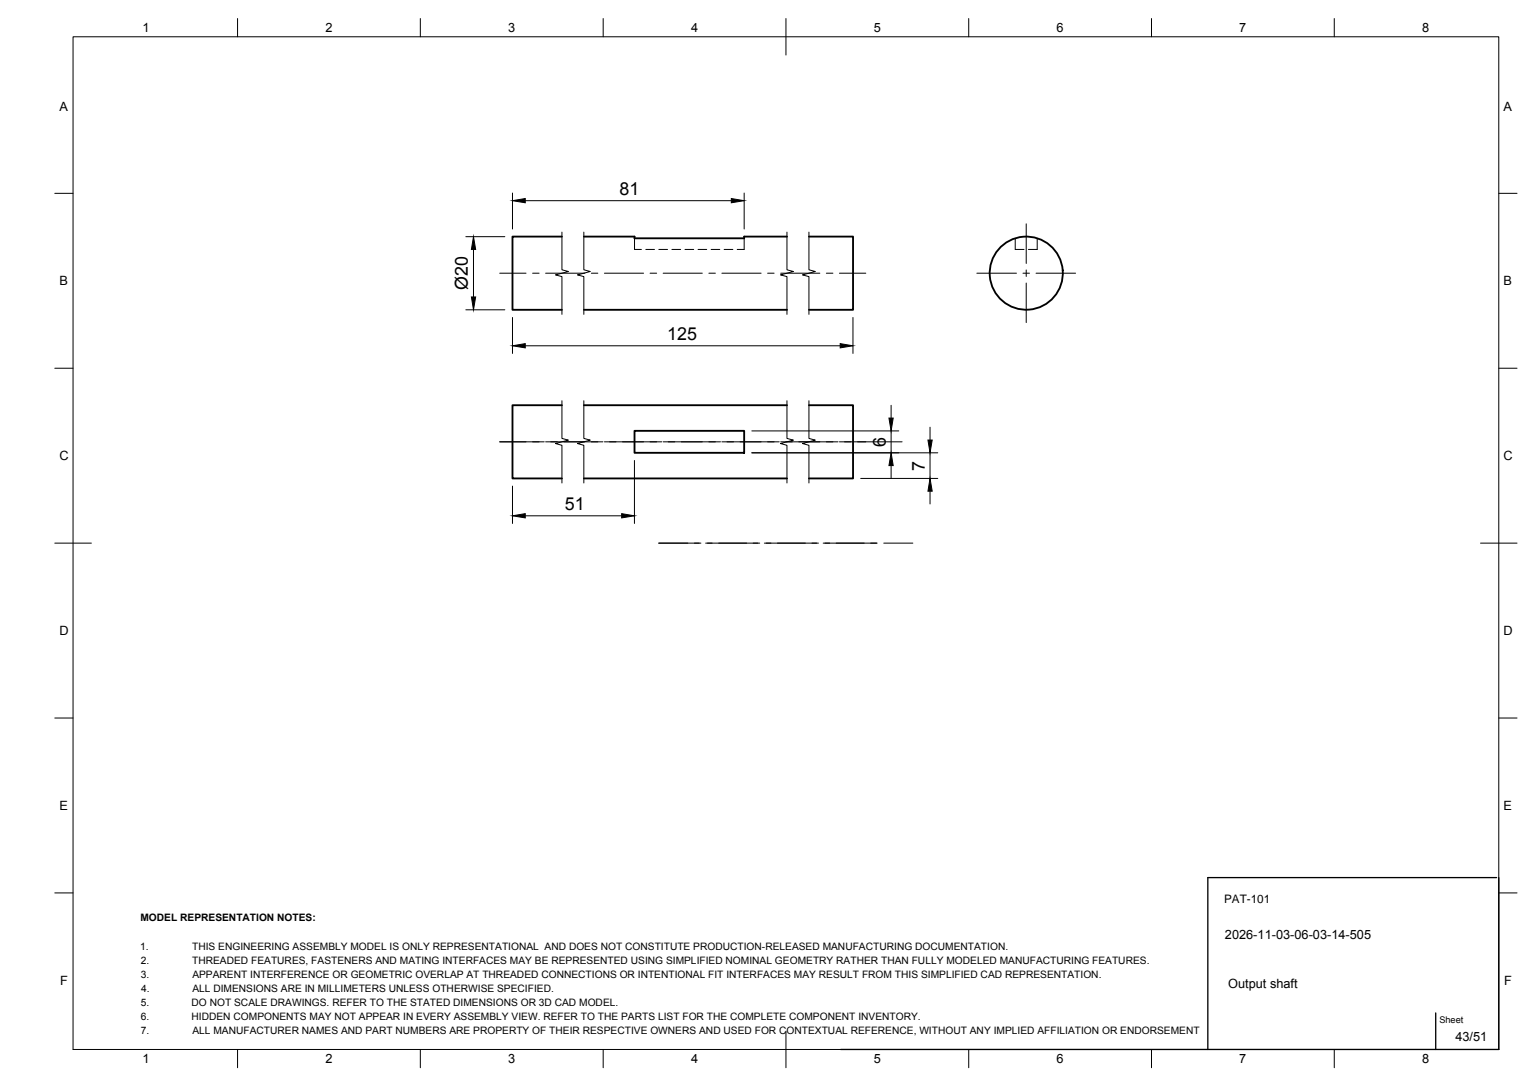
ISO-10303-21;
HEADER;
/* Generated by software containing ST-Developer
 * from STEP Tools, Inc. (www.steptools.com) 
 */

FILE_DESCRIPTION(
/* description */ ('Spur gear reduction stage 2-1 on bearing plates'),
/* implementation_level */ '2;1');

FILE_NAME(
/* name */ 'Output shaft.step',
/* time_stamp */ '2026-10-28T03:22:07-07:00',
/* author */ (''),
/* organization */ (''),
/* preprocessor_version */ 'ST-DEVELOPER v20.2',
/* originating_system */ 'Autodesk Translation Framework v15.17.0.0',
/* authorisation */ '');

FILE_SCHEMA (('AUTOMOTIVE_DESIGN { 1 0 10303 214 3 1 1 }'));
ENDSEC;

DATA;
#10=MECHANICAL_DESIGN_GEOMETRIC_PRESENTATION_REPRESENTATION('',(#995),#53909);
#894=SHAPE_REPRESENTATION_RELATIONSHIP('SRR','None',#54125,#937);
#937=ADVANCED_BREP_SHAPE_REPRESENTATION('',(#1050),#53899);
#995=STYLED_ITEM('',(#54397),#1050);
#1050=MANIFOLD_SOLID_BREP('Body1',#11322);
#1217=FACE_BOUND('',#2734,.T.);
#1415=PLANE('',#12678);
#1416=PLANE('',#12679);
#1417=PLANE('',#12681);
#1418=PLANE('',#12682);
#1419=PLANE('',#12683);
#1420=PLANE('',#12688);
#1421=PLANE('',#12689);
#1923=FACE_OUTER_BOUND('',#2728,.T.);
#1924=FACE_OUTER_BOUND('',#2729,.T.);
#1925=FACE_OUTER_BOUND('',#2730,.T.);
#1926=FACE_OUTER_BOUND('',#2731,.T.);
#1927=FACE_OUTER_BOUND('',#2732,.T.);
#1928=FACE_OUTER_BOUND('',#2733,.T.);
#1929=FACE_OUTER_BOUND('',#2735,.T.);
#1930=FACE_OUTER_BOUND('',#2736,.T.);
#2728=EDGE_LOOP('',(#9190,#9191,#9192,#9193));
#2729=EDGE_LOOP('',(#9194,#9195,#9196,#9197));
#2730=EDGE_LOOP('',(#9198,#9199,#9200,#9201));
#2731=EDGE_LOOP('',(#9202,#9203,#9204,#9205));
#2732=EDGE_LOOP('',(#9206,#9207,#9208,#9209));
#2733=EDGE_LOOP('',(#9210,#9211,#9212,#9213));
#2734=EDGE_LOOP('',(#9214,#9215,#9216,#9217));
#2735=EDGE_LOOP('',(#9218));
#2736=EDGE_LOOP('',(#9219));
#3373=LINE('',#29846,#4014);
#3374=LINE('',#29848,#4015);
#3375=LINE('',#29850,#4016);
#3376=LINE('',#29851,#4017);
#3377=LINE('',#29856,#4018);
#3378=LINE('',#29857,#4019);
#3379=LINE('',#29860,#4020);
#3380=LINE('',#29862,#4021);
#3381=LINE('',#29863,#4022);
#3382=LINE('',#29865,#4023);
#3383=LINE('',#29872,#4024);
#4014=VECTOR('',#15124,1.);
#4015=VECTOR('',#15125,1.);
#4016=VECTOR('',#15126,1.);
#4017=VECTOR('',#15127,1.);
#4018=VECTOR('',#15132,1.);
#4019=VECTOR('',#15133,1.);
#4020=VECTOR('',#15136,1.);
#4021=VECTOR('',#15137,1.);
#4022=VECTOR('',#15138,1.);
#4023=VECTOR('',#15141,1.);
#4024=VECTOR('',#15150,1.);
#4662=CIRCLE('',#12680,1.);
#4663=CIRCLE('',#12684,1.);
#4664=CIRCLE('',#12686,1.);
#4665=CIRCLE('',#12687,1.);
#5408=VERTEX_POINT('',#29844);
#5409=VERTEX_POINT('',#29845);
#5410=VERTEX_POINT('',#29847);
#5411=VERTEX_POINT('',#29849);
#5412=VERTEX_POINT('',#29853);
#5413=VERTEX_POINT('',#29855);
#5414=VERTEX_POINT('',#29859);
#5415=VERTEX_POINT('',#29861);
#5416=VERTEX_POINT('',#29869);
#5417=VERTEX_POINT('',#29871);
#6737=EDGE_CURVE('',#5408,#5409,#3373,.T.);
#6738=EDGE_CURVE('',#5408,#5410,#3374,.T.);
#6739=EDGE_CURVE('',#5411,#5410,#3375,.T.);
#6740=EDGE_CURVE('',#5411,#5409,#3376,.T.);
#6741=EDGE_CURVE('',#5409,#5412,#4662,.T.);
#6742=EDGE_CURVE('',#5413,#5411,#3377,.T.);
#6743=EDGE_CURVE('',#5412,#5413,#3378,.T.);
#6744=EDGE_CURVE('',#5412,#5414,#3379,.T.);
#6745=EDGE_CURVE('',#5413,#5415,#3380,.T.);
#6746=EDGE_CURVE('',#5415,#5414,#3381,.T.);
#6747=EDGE_CURVE('',#5410,#5415,#3382,.T.);
#6748=EDGE_CURVE('',#5414,#5408,#4663,.T.);
#6749=EDGE_CURVE('',#5416,#5416,#4664,.T.);
#6750=EDGE_CURVE('',#5416,#5417,#3383,.T.);
#6751=EDGE_CURVE('',#5417,#5417,#4665,.T.);
#9190=ORIENTED_EDGE('',*,*,#6737,.F.);
#9191=ORIENTED_EDGE('',*,*,#6738,.T.);
#9192=ORIENTED_EDGE('',*,*,#6739,.F.);
#9193=ORIENTED_EDGE('',*,*,#6740,.T.);
#9194=ORIENTED_EDGE('',*,*,#6741,.F.);
#9195=ORIENTED_EDGE('',*,*,#6740,.F.);
#9196=ORIENTED_EDGE('',*,*,#6742,.F.);
#9197=ORIENTED_EDGE('',*,*,#6743,.F.);
#9198=ORIENTED_EDGE('',*,*,#6744,.F.);
#9199=ORIENTED_EDGE('',*,*,#6743,.T.);
#9200=ORIENTED_EDGE('',*,*,#6745,.T.);
#9201=ORIENTED_EDGE('',*,*,#6746,.T.);
#9202=ORIENTED_EDGE('',*,*,#6742,.T.);
#9203=ORIENTED_EDGE('',*,*,#6739,.T.);
#9204=ORIENTED_EDGE('',*,*,#6747,.T.);
#9205=ORIENTED_EDGE('',*,*,#6745,.F.);
#9206=ORIENTED_EDGE('',*,*,#6748,.F.);
#9207=ORIENTED_EDGE('',*,*,#6746,.F.);
#9208=ORIENTED_EDGE('',*,*,#6747,.F.);
#9209=ORIENTED_EDGE('',*,*,#6738,.F.);
#9210=ORIENTED_EDGE('',*,*,#6749,.F.);
#9211=ORIENTED_EDGE('',*,*,#6750,.T.);
#9212=ORIENTED_EDGE('',*,*,#6751,.T.);
#9213=ORIENTED_EDGE('',*,*,#6750,.F.);
#9214=ORIENTED_EDGE('',*,*,#6744,.T.);
#9215=ORIENTED_EDGE('',*,*,#6748,.T.);
#9216=ORIENTED_EDGE('',*,*,#6737,.T.);
#9217=ORIENTED_EDGE('',*,*,#6741,.T.);
#9218=ORIENTED_EDGE('',*,*,#6749,.T.);
#9219=ORIENTED_EDGE('',*,*,#6751,.F.);
#10565=CYLINDRICAL_SURFACE('',#12685,1.);
#11043=ADVANCED_FACE('',(#1923),#1415,.F.);
#11044=ADVANCED_FACE('',(#1924),#1416,.T.);
#11045=ADVANCED_FACE('',(#1925),#1417,.F.);
#11046=ADVANCED_FACE('',(#1926),#1418,.F.);
#11047=ADVANCED_FACE('',(#1927),#1419,.F.);
#11048=ADVANCED_FACE('',(#1928,#1217),#10565,.T.);
#11049=ADVANCED_FACE('',(#1929),#1420,.T.);
#11050=ADVANCED_FACE('',(#1930),#1421,.F.);
#11322=CLOSED_SHELL('',(#11043,#11044,#11045,#11046,#11047,#11048,#11049,
#11050));
#12677=AXIS2_PLACEMENT_3D('',#29842,#15120,#15121);
#12678=AXIS2_PLACEMENT_3D('',#29843,#15122,#15123);
#12679=AXIS2_PLACEMENT_3D('',#29852,#15128,#15129);
#12680=AXIS2_PLACEMENT_3D('',#29854,#15130,#15131);
#12681=AXIS2_PLACEMENT_3D('',#29858,#15134,#15135);
#12682=AXIS2_PLACEMENT_3D('',#29864,#15139,#15140);
#12683=AXIS2_PLACEMENT_3D('',#29866,#15142,#15143);
#12684=AXIS2_PLACEMENT_3D('',#29867,#15144,#15145);
#12685=AXIS2_PLACEMENT_3D('',#29868,#15146,#15147);
#12686=AXIS2_PLACEMENT_3D('',#29870,#15148,#15149);
#12687=AXIS2_PLACEMENT_3D('',#29873,#15151,#15152);
#12688=AXIS2_PLACEMENT_3D('',#29874,#15153,#15154);
#12689=AXIS2_PLACEMENT_3D('',#29875,#15155,#15156);
#15120=DIRECTION('axis',(0.,0.,1.));
#15121=DIRECTION('refdir',(1.,0.,0.));
#15122=DIRECTION('center_axis',(-1.,0.,0.));
#15123=DIRECTION('ref_axis',(0.,0.,1.));
#15124=DIRECTION('',(0.,-1.,0.));
#15125=DIRECTION('',(0.,0.,1.));
#15126=DIRECTION('',(0.,1.,0.));
#15127=DIRECTION('',(0.,0.,-1.));
#15128=DIRECTION('center_axis',(0.,1.,0.));
#15129=DIRECTION('ref_axis',(1.,0.,0.));
#15130=DIRECTION('center_axis',(0.,-1.,0.));
#15131=DIRECTION('ref_axis',(1.,0.,0.));
#15132=DIRECTION('',(-1.,0.,0.));
#15133=DIRECTION('',(0.,0.,1.));
#15134=DIRECTION('center_axis',(1.,0.,0.));
#15135=DIRECTION('ref_axis',(0.,0.,-1.));
#15136=DIRECTION('',(0.,1.,0.));
#15137=DIRECTION('',(0.,1.,0.));
#15138=DIRECTION('',(0.,0.,-1.));
#15139=DIRECTION('center_axis',(0.,0.,1.));
#15140=DIRECTION('ref_axis',(1.,0.,0.));
#15141=DIRECTION('',(1.,0.,0.));
#15142=DIRECTION('center_axis',(0.,1.,0.));
#15143=DIRECTION('ref_axis',(0.,0.,1.));
#15144=DIRECTION('center_axis',(0.,1.,0.));
#15145=DIRECTION('ref_axis',(1.,0.,0.));
#15146=DIRECTION('center_axis',(0.,1.,0.));
#15147=DIRECTION('ref_axis',(1.,0.,0.));
#15148=DIRECTION('center_axis',(0.,1.,0.));
#15149=DIRECTION('ref_axis',(1.,0.,0.));
#15150=DIRECTION('',(0.,-1.,0.));
#15151=DIRECTION('center_axis',(0.,1.,0.));
#15152=DIRECTION('ref_axis',(1.,0.,0.));
#15153=DIRECTION('center_axis',(0.,1.,0.));
#15154=DIRECTION('ref_axis',(1.,0.,0.));
#15155=DIRECTION('center_axis',(0.,1.,0.));
#15156=DIRECTION('ref_axis',(1.,0.,0.));
#29842=CARTESIAN_POINT('',(0.,0.,0.));
#29843=CARTESIAN_POINT('Origin',(-0.3,-0.9,-1.1));
#29844=CARTESIAN_POINT('',(-0.3,2.1,-0.953939201416946));
#29845=CARTESIAN_POINT('',(-0.3,-0.9,-0.953939201416946));
#29846=CARTESIAN_POINT('',(-0.3,-6.,-0.953939201416946));
#29847=CARTESIAN_POINT('',(-0.3,2.1,-0.65));
#29848=CARTESIAN_POINT('',(-0.3,2.1,-0.65));
#29849=CARTESIAN_POINT('',(-0.3,-0.9,-0.65));
#29850=CARTESIAN_POINT('',(-0.3,-0.9,-0.65));
#29851=CARTESIAN_POINT('',(-0.3,-0.9,-0.65));
#29852=CARTESIAN_POINT('Origin',(0.,-0.9,-0.875));
#29853=CARTESIAN_POINT('',(0.3,-0.9,-0.953939201416946));
#29854=CARTESIAN_POINT('Origin',(0.,-0.9,0.));
#29855=CARTESIAN_POINT('',(0.3,-0.9,-0.65));
#29856=CARTESIAN_POINT('',(0.3,-0.9,-0.65));
#29857=CARTESIAN_POINT('',(0.3,-0.9,-1.1));
#29858=CARTESIAN_POINT('Origin',(0.3,-0.9,-0.65));
#29859=CARTESIAN_POINT('',(0.3,2.1,-0.953939201416946));
#29860=CARTESIAN_POINT('',(0.3,-6.,-0.953939201416946));
#29861=CARTESIAN_POINT('',(0.3,2.1,-0.65));
#29862=CARTESIAN_POINT('',(0.3,-0.9,-0.65));
#29863=CARTESIAN_POINT('',(0.3,2.1,-1.1));
#29864=CARTESIAN_POINT('Origin',(-0.3,-0.9,-0.65));
#29865=CARTESIAN_POINT('',(0.3,2.1,-0.65));
#29866=CARTESIAN_POINT('Origin',(0.,2.1,-0.875));
#29867=CARTESIAN_POINT('Origin',(0.,2.1,0.));
#29868=CARTESIAN_POINT('Origin',(0.,-6.,0.));
#29869=CARTESIAN_POINT('',(-1.,6.5,1.22464679914735E-16));
#29870=CARTESIAN_POINT('Origin',(0.,6.5,0.));
#29871=CARTESIAN_POINT('',(-1.,-6.,1.22464679914735E-16));
#29872=CARTESIAN_POINT('',(-1.,-6.,1.22464679914735E-16));
#29873=CARTESIAN_POINT('Origin',(0.,-6.,0.));
#29874=CARTESIAN_POINT('Origin',(0.,6.5,0.));
#29875=CARTESIAN_POINT('Origin',(0.,-6.,0.));
#53849=UNCERTAINTY_MEASURE_WITH_UNIT(LENGTH_MEASURE(0.001),#53910,
'DISTANCE_ACCURACY_VALUE',
'Maximum model space distance between geometric entities at asserted c
onnectivities');
#53859=UNCERTAINTY_MEASURE_WITH_UNIT(LENGTH_MEASURE(0.001),#53910,
'DISTANCE_ACCURACY_VALUE',
'Maximum model space distance between geometric entities at asserted c
onnectivities');
#53899=(
GEOMETRIC_REPRESENTATION_CONTEXT(3)
GLOBAL_UNCERTAINTY_ASSIGNED_CONTEXT((#53849))
GLOBAL_UNIT_ASSIGNED_CONTEXT((#53910,#53912,#53913))
REPRESENTATION_CONTEXT('','3D')
);
#53909=(
GEOMETRIC_REPRESENTATION_CONTEXT(3)
GLOBAL_UNCERTAINTY_ASSIGNED_CONTEXT((#53859))
GLOBAL_UNIT_ASSIGNED_CONTEXT((#53910,#53912,#53913))
REPRESENTATION_CONTEXT('','3D')
);
#53910=(
LENGTH_UNIT()
NAMED_UNIT(*)
SI_UNIT(.CENTI.,.METRE.)
);
#53912=(
NAMED_UNIT(*)
PLANE_ANGLE_UNIT()
SI_UNIT($,.RADIAN.)
);
#53913=(
NAMED_UNIT(*)
SI_UNIT($,.STERADIAN.)
SOLID_ANGLE_UNIT()
);
#53953=SHAPE_DEFINITION_REPRESENTATION(#54051,#54125);
#54051=PRODUCT_DEFINITION_SHAPE('',$,#54175);
#54125=SHAPE_REPRESENTATION('',(#12677),#53899);
#54135=PRODUCT_DEFINITION_CONTEXT('part definition',#54284,'design');
#54175=PRODUCT_DEFINITION('Output shaft','Output shaft',#54224,#54135);
#54224=PRODUCT_DEFINITION_FORMATION('',$,#54325);
#54284=APPLICATION_CONTEXT(
'Core Data for Automotive Mechanical Design Process');
#54285=PRODUCT_CONTEXT('part definition',#54284,'mechanical');
#54325=PRODUCT('Output shaft','Output shaft','Output shaft',(#54285));
#54391=COLOUR_RGB('Grey',0.48,0.52,0.57);
#54392=FILL_AREA_STYLE_COLOUR('',#54391);
#54393=FILL_AREA_STYLE('',(#54392));
#54394=SURFACE_STYLE_FILL_AREA(#54393);
#54395=SURFACE_SIDE_STYLE('',(#54394));
#54396=SURFACE_STYLE_USAGE(.BOTH.,#54395);
#54397=PRESENTATION_STYLE_ASSIGNMENT((#54396));
ENDSEC;
END-ISO-10303-21;
